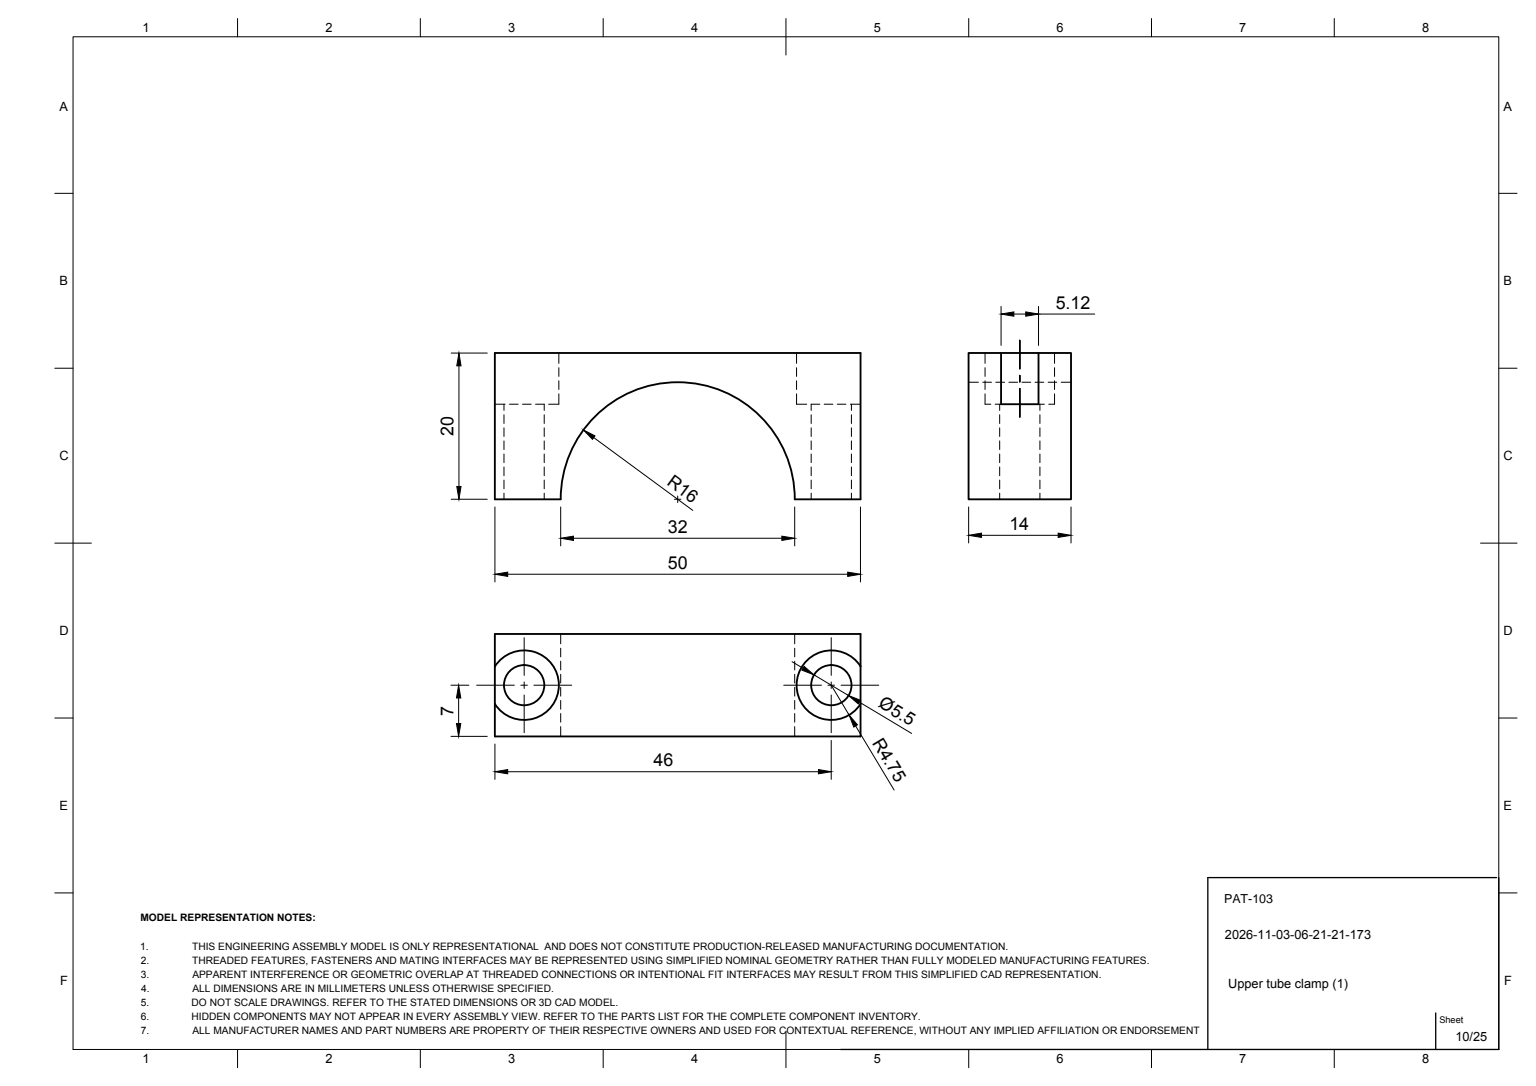
ISO-10303-21;
HEADER;
/* Generated by software containing ST-Developer
 * from STEP Tools, Inc. (www.steptools.com) 
 */

FILE_DESCRIPTION(
/* description */ ('Telescoping shaft support with lock collar'),
/* implementation_level */ '2;1');

FILE_NAME(
/* name */ 'Upper tube clamp (1).step',
/* time_stamp */ '2026-10-27T10:48:51-07:00',
/* author */ (''),
/* organization */ (''),
/* preprocessor_version */ 'ST-DEVELOPER v20.2',
/* originating_system */ 'Autodesk Translation Framework v15.17.0.0',
/* authorisation */ '');

FILE_SCHEMA (('AUTOMOTIVE_DESIGN { 1 0 10303 214 3 1 1 }'));
ENDSEC;

DATA;
#10=MECHANICAL_DESIGN_GEOMETRIC_PRESENTATION_REPRESENTATION('',(#246),#7349);
#206=SHAPE_REPRESENTATION_RELATIONSHIP('SRR','None',#7448,#226);
#226=ADVANCED_BREP_SHAPE_REPRESENTATION('',(#266),#7332);
#246=STYLED_ITEM('',(#7641),#266);
#266=MANIFOLD_SOLID_BREP('Body1',#3969);
#309=FACE_BOUND('',#828,.T.);
#310=FACE_BOUND('',#831,.T.);
#311=FACE_BOUND('',#840,.T.);
#312=FACE_BOUND('',#844,.T.);
#406=PLANE('',#4373);
#407=PLANE('',#4378);
#408=PLANE('',#4383);
#409=PLANE('',#4384);
#410=PLANE('',#4392);
#411=PLANE('',#4393);
#412=PLANE('',#4394);
#413=PLANE('',#4395);
#414=PLANE('',#4396);
#571=FACE_OUTER_BOUND('',#827,.T.);
#572=FACE_OUTER_BOUND('',#829,.T.);
#573=FACE_OUTER_BOUND('',#830,.T.);
#574=FACE_OUTER_BOUND('',#832,.T.);
#575=FACE_OUTER_BOUND('',#833,.T.);
#576=FACE_OUTER_BOUND('',#834,.T.);
#577=FACE_OUTER_BOUND('',#835,.T.);
#578=FACE_OUTER_BOUND('',#836,.T.);
#579=FACE_OUTER_BOUND('',#837,.T.);
#580=FACE_OUTER_BOUND('',#838,.T.);
#581=FACE_OUTER_BOUND('',#839,.T.);
#582=FACE_OUTER_BOUND('',#841,.T.);
#583=FACE_OUTER_BOUND('',#842,.T.);
#584=FACE_OUTER_BOUND('',#843,.T.);
#827=EDGE_LOOP('',(#3014,#3015));
#828=EDGE_LOOP('',(#3016));
#829=EDGE_LOOP('',(#3017,#3018,#3019,#3020));
#830=EDGE_LOOP('',(#3021,#3022));
#831=EDGE_LOOP('',(#3023));
#832=EDGE_LOOP('',(#3024,#3025,#3026,#3027));
#833=EDGE_LOOP('',(#3028,#3029,#3030,#3031,#3032,#3033,#3034,#3035));
#834=EDGE_LOOP('',(#3036,#3037,#3038,#3039,#3040,#3041,#3042,#3043));
#835=EDGE_LOOP('',(#3044,#3045,#3046,#3047));
#836=EDGE_LOOP('',(#3048,#3049,#3050,#3051));
#837=EDGE_LOOP('',(#3052,#3053,#3054,#3055));
#838=EDGE_LOOP('',(#3056,#3057,#3058,#3059,#3060,#3061));
#839=EDGE_LOOP('',(#3062,#3063,#3064,#3065));
#840=EDGE_LOOP('',(#3066));
#841=EDGE_LOOP('',(#3067,#3068,#3069,#3070,#3071,#3072));
#842=EDGE_LOOP('',(#3073,#3074,#3075,#3076,#3077,#3078,#3079,#3080));
#843=EDGE_LOOP('',(#3081,#3082,#3083,#3084));
#844=EDGE_LOOP('',(#3085));
#1131=LINE('',#6384,#1411);
#1132=LINE('',#6390,#1412);
#1133=LINE('',#6393,#1413);
#1134=LINE('',#6397,#1414);
#1135=LINE('',#6403,#1415);
#1136=LINE('',#6406,#1416);
#1137=LINE('',#6409,#1417);
#1138=LINE('',#6411,#1418);
#1139=LINE('',#6413,#1419);
#1140=LINE('',#6415,#1420);
#1141=LINE('',#6416,#1421);
#1142=LINE('',#6419,#1422);
#1143=LINE('',#6421,#1423);
#1144=LINE('',#6423,#1424);
#1145=LINE('',#6425,#1425);
#1146=LINE('',#6426,#1426);
#1147=LINE('',#6430,#1427);
#1148=LINE('',#6434,#1428);
#1149=LINE('',#6440,#1429);
#1150=LINE('',#6443,#1430);
#1151=LINE('',#6445,#1431);
#1152=LINE('',#6446,#1432);
#1153=LINE('',#6447,#1433);
#1154=LINE('',#6449,#1434);
#1155=LINE('',#6451,#1435);
#1156=LINE('',#6452,#1436);
#1411=VECTOR('',#5145,1.);
#1412=VECTOR('',#5152,1.);
#1413=VECTOR('',#5155,1.);
#1414=VECTOR('',#5158,1.);
#1415=VECTOR('',#5165,1.);
#1416=VECTOR('',#5168,1.);
#1417=VECTOR('',#5171,1.);
#1418=VECTOR('',#5172,1.);
#1419=VECTOR('',#5173,1.);
#1420=VECTOR('',#5174,1.);
#1421=VECTOR('',#5175,1.);
#1422=VECTOR('',#5178,1.);
#1423=VECTOR('',#5179,1.);
#1424=VECTOR('',#5180,1.);
#1425=VECTOR('',#5181,1.);
#1426=VECTOR('',#5182,1.);
#1427=VECTOR('',#5187,0.274999999999999);
#1428=VECTOR('',#5192,0.274999999999999);
#1429=VECTOR('',#5197,1.);
#1430=VECTOR('',#5200,1.);
#1431=VECTOR('',#5203,1.);
#1432=VECTOR('',#5204,1.);
#1433=VECTOR('',#5205,1.);
#1434=VECTOR('',#5208,1.);
#1435=VECTOR('',#5211,1.);
#1436=VECTOR('',#5212,1.);
#1669=CIRCLE('',#4374,0.475000000000001);
#1670=CIRCLE('',#4375,0.274999999999999);
#1671=CIRCLE('',#4377,0.475000000000001);
#1672=CIRCLE('',#4379,0.475000000000001);
#1673=CIRCLE('',#4380,0.274999999999999);
#1674=CIRCLE('',#4382,0.475000000000001);
#1675=CIRCLE('',#4386,0.274999999999999);
#1676=CIRCLE('',#4388,0.274999999999999);
#1677=CIRCLE('',#4390,1.6);
#1678=CIRCLE('',#4391,1.6);
#1922=VERTEX_POINT('',#6382);
#1923=VERTEX_POINT('',#6383);
#1924=VERTEX_POINT('',#6386);
#1925=VERTEX_POINT('',#6389);
#1926=VERTEX_POINT('',#6391);
#1927=VERTEX_POINT('',#6395);
#1928=VERTEX_POINT('',#6396);
#1929=VERTEX_POINT('',#6399);
#1930=VERTEX_POINT('',#6402);
#1931=VERTEX_POINT('',#6404);
#1932=VERTEX_POINT('',#6408);
#1933=VERTEX_POINT('',#6410);
#1934=VERTEX_POINT('',#6412);
#1935=VERTEX_POINT('',#6414);
#1936=VERTEX_POINT('',#6418);
#1937=VERTEX_POINT('',#6420);
#1938=VERTEX_POINT('',#6422);
#1939=VERTEX_POINT('',#6424);
#1940=VERTEX_POINT('',#6428);
#1941=VERTEX_POINT('',#6432);
#1942=VERTEX_POINT('',#6436);
#1943=VERTEX_POINT('',#6437);
#1944=VERTEX_POINT('',#6439);
#1945=VERTEX_POINT('',#6441);
#2319=EDGE_CURVE('',#1922,#1923,#1131,.T.);
#2320=EDGE_CURVE('',#1922,#1923,#1669,.T.);
#2321=EDGE_CURVE('',#1924,#1924,#1670,.T.);
#2322=EDGE_CURVE('',#1925,#1922,#1132,.T.);
#2323=EDGE_CURVE('',#1926,#1925,#1671,.T.);
#2324=EDGE_CURVE('',#1923,#1926,#1133,.T.);
#2325=EDGE_CURVE('',#1927,#1928,#1134,.T.);
#2326=EDGE_CURVE('',#1927,#1928,#1672,.T.);
#2327=EDGE_CURVE('',#1929,#1929,#1673,.T.);
#2328=EDGE_CURVE('',#1930,#1927,#1135,.T.);
#2329=EDGE_CURVE('',#1931,#1930,#1674,.T.);
#2330=EDGE_CURVE('',#1928,#1931,#1136,.T.);
#2331=EDGE_CURVE('',#1932,#1926,#1137,.T.);
#2332=EDGE_CURVE('',#1933,#1932,#1138,.T.);
#2333=EDGE_CURVE('',#1933,#1934,#1139,.T.);
#2334=EDGE_CURVE('',#1934,#1935,#1140,.T.);
#2335=EDGE_CURVE('',#1925,#1935,#1141,.T.);
#2336=EDGE_CURVE('',#1936,#1931,#1142,.T.);
#2337=EDGE_CURVE('',#1937,#1936,#1143,.T.);
#2338=EDGE_CURVE('',#1937,#1938,#1144,.T.);
#2339=EDGE_CURVE('',#1938,#1939,#1145,.T.);
#2340=EDGE_CURVE('',#1930,#1939,#1146,.T.);
#2341=EDGE_CURVE('',#1940,#1940,#1675,.T.);
#2342=EDGE_CURVE('',#1940,#1924,#1147,.T.);
#2343=EDGE_CURVE('',#1941,#1941,#1676,.T.);
#2344=EDGE_CURVE('',#1941,#1929,#1148,.T.);
#2345=EDGE_CURVE('',#1942,#1943,#1677,.T.);
#2346=EDGE_CURVE('',#1944,#1942,#1149,.T.);
#2347=EDGE_CURVE('',#1945,#1944,#1678,.T.);
#2348=EDGE_CURVE('',#1943,#1945,#1150,.T.);
#2349=EDGE_CURVE('',#1944,#1937,#1151,.T.);
#2350=EDGE_CURVE('',#1935,#1936,#1152,.T.);
#2351=EDGE_CURVE('',#1934,#1945,#1153,.T.);
#2352=EDGE_CURVE('',#1938,#1942,#1154,.T.);
#2353=EDGE_CURVE('',#1943,#1933,#1155,.T.);
#2354=EDGE_CURVE('',#1939,#1932,#1156,.T.);
#3014=ORIENTED_EDGE('',*,*,#2319,.F.);
#3015=ORIENTED_EDGE('',*,*,#2320,.T.);
#3016=ORIENTED_EDGE('',*,*,#2321,.F.);
#3017=ORIENTED_EDGE('',*,*,#2322,.F.);
#3018=ORIENTED_EDGE('',*,*,#2323,.F.);
#3019=ORIENTED_EDGE('',*,*,#2324,.F.);
#3020=ORIENTED_EDGE('',*,*,#2320,.F.);
#3021=ORIENTED_EDGE('',*,*,#2325,.F.);
#3022=ORIENTED_EDGE('',*,*,#2326,.T.);
#3023=ORIENTED_EDGE('',*,*,#2327,.F.);
#3024=ORIENTED_EDGE('',*,*,#2328,.F.);
#3025=ORIENTED_EDGE('',*,*,#2329,.F.);
#3026=ORIENTED_EDGE('',*,*,#2330,.F.);
#3027=ORIENTED_EDGE('',*,*,#2326,.F.);
#3028=ORIENTED_EDGE('',*,*,#2322,.T.);
#3029=ORIENTED_EDGE('',*,*,#2319,.T.);
#3030=ORIENTED_EDGE('',*,*,#2324,.T.);
#3031=ORIENTED_EDGE('',*,*,#2331,.F.);
#3032=ORIENTED_EDGE('',*,*,#2332,.F.);
#3033=ORIENTED_EDGE('',*,*,#2333,.T.);
#3034=ORIENTED_EDGE('',*,*,#2334,.T.);
#3035=ORIENTED_EDGE('',*,*,#2335,.F.);
#3036=ORIENTED_EDGE('',*,*,#2328,.T.);
#3037=ORIENTED_EDGE('',*,*,#2325,.T.);
#3038=ORIENTED_EDGE('',*,*,#2330,.T.);
#3039=ORIENTED_EDGE('',*,*,#2336,.F.);
#3040=ORIENTED_EDGE('',*,*,#2337,.F.);
#3041=ORIENTED_EDGE('',*,*,#2338,.T.);
#3042=ORIENTED_EDGE('',*,*,#2339,.T.);
#3043=ORIENTED_EDGE('',*,*,#2340,.F.);
#3044=ORIENTED_EDGE('',*,*,#2341,.F.);
#3045=ORIENTED_EDGE('',*,*,#2342,.T.);
#3046=ORIENTED_EDGE('',*,*,#2321,.T.);
#3047=ORIENTED_EDGE('',*,*,#2342,.F.);
#3048=ORIENTED_EDGE('',*,*,#2343,.F.);
#3049=ORIENTED_EDGE('',*,*,#2344,.T.);
#3050=ORIENTED_EDGE('',*,*,#2327,.T.);
#3051=ORIENTED_EDGE('',*,*,#2344,.F.);
#3052=ORIENTED_EDGE('',*,*,#2345,.F.);
#3053=ORIENTED_EDGE('',*,*,#2346,.F.);
#3054=ORIENTED_EDGE('',*,*,#2347,.F.);
#3055=ORIENTED_EDGE('',*,*,#2348,.F.);
#3056=ORIENTED_EDGE('',*,*,#2347,.T.);
#3057=ORIENTED_EDGE('',*,*,#2349,.T.);
#3058=ORIENTED_EDGE('',*,*,#2337,.T.);
#3059=ORIENTED_EDGE('',*,*,#2350,.F.);
#3060=ORIENTED_EDGE('',*,*,#2334,.F.);
#3061=ORIENTED_EDGE('',*,*,#2351,.T.);
#3062=ORIENTED_EDGE('',*,*,#2346,.T.);
#3063=ORIENTED_EDGE('',*,*,#2352,.F.);
#3064=ORIENTED_EDGE('',*,*,#2338,.F.);
#3065=ORIENTED_EDGE('',*,*,#2349,.F.);
#3066=ORIENTED_EDGE('',*,*,#2343,.T.);
#3067=ORIENTED_EDGE('',*,*,#2345,.T.);
#3068=ORIENTED_EDGE('',*,*,#2353,.T.);
#3069=ORIENTED_EDGE('',*,*,#2332,.T.);
#3070=ORIENTED_EDGE('',*,*,#2354,.F.);
#3071=ORIENTED_EDGE('',*,*,#2339,.F.);
#3072=ORIENTED_EDGE('',*,*,#2352,.T.);
#3073=ORIENTED_EDGE('',*,*,#2323,.T.);
#3074=ORIENTED_EDGE('',*,*,#2335,.T.);
#3075=ORIENTED_EDGE('',*,*,#2350,.T.);
#3076=ORIENTED_EDGE('',*,*,#2336,.T.);
#3077=ORIENTED_EDGE('',*,*,#2329,.T.);
#3078=ORIENTED_EDGE('',*,*,#2340,.T.);
#3079=ORIENTED_EDGE('',*,*,#2354,.T.);
#3080=ORIENTED_EDGE('',*,*,#2331,.T.);
#3081=ORIENTED_EDGE('',*,*,#2348,.T.);
#3082=ORIENTED_EDGE('',*,*,#2351,.F.);
#3083=ORIENTED_EDGE('',*,*,#2333,.F.);
#3084=ORIENTED_EDGE('',*,*,#2353,.F.);
#3085=ORIENTED_EDGE('',*,*,#2341,.T.);
#3689=CYLINDRICAL_SURFACE('',#4376,0.475000000000001);
#3690=CYLINDRICAL_SURFACE('',#4381,0.475000000000001);
#3691=CYLINDRICAL_SURFACE('',#4385,0.274999999999999);
#3692=CYLINDRICAL_SURFACE('',#4387,0.274999999999999);
#3693=CYLINDRICAL_SURFACE('',#4389,1.6);
#3814=ADVANCED_FACE('',(#571,#309),#406,.T.);
#3815=ADVANCED_FACE('',(#572),#3689,.F.);
#3816=ADVANCED_FACE('',(#573,#310),#407,.T.);
#3817=ADVANCED_FACE('',(#574),#3690,.F.);
#3818=ADVANCED_FACE('',(#575),#408,.T.);
#3819=ADVANCED_FACE('',(#576),#409,.T.);
#3820=ADVANCED_FACE('',(#577),#3691,.F.);
#3821=ADVANCED_FACE('',(#578),#3692,.F.);
#3822=ADVANCED_FACE('',(#579),#3693,.F.);
#3823=ADVANCED_FACE('',(#580),#410,.T.);
#3824=ADVANCED_FACE('',(#581,#311),#411,.F.);
#3825=ADVANCED_FACE('',(#582),#412,.T.);
#3826=ADVANCED_FACE('',(#583),#413,.T.);
#3827=ADVANCED_FACE('',(#584,#312),#414,.F.);
#3969=CLOSED_SHELL('',(#3814,#3815,#3816,#3817,#3818,#3819,#3820,#3821,
#3822,#3823,#3824,#3825,#3826,#3827));
#4372=AXIS2_PLACEMENT_3D('',#6380,#5141,#5142);
#4373=AXIS2_PLACEMENT_3D('',#6381,#5143,#5144);
#4374=AXIS2_PLACEMENT_3D('',#6385,#5146,#5147);
#4375=AXIS2_PLACEMENT_3D('',#6387,#5148,#5149);
#4376=AXIS2_PLACEMENT_3D('',#6388,#5150,#5151);
#4377=AXIS2_PLACEMENT_3D('',#6392,#5153,#5154);
#4378=AXIS2_PLACEMENT_3D('',#6394,#5156,#5157);
#4379=AXIS2_PLACEMENT_3D('',#6398,#5159,#5160);
#4380=AXIS2_PLACEMENT_3D('',#6400,#5161,#5162);
#4381=AXIS2_PLACEMENT_3D('',#6401,#5163,#5164);
#4382=AXIS2_PLACEMENT_3D('',#6405,#5166,#5167);
#4383=AXIS2_PLACEMENT_3D('',#6407,#5169,#5170);
#4384=AXIS2_PLACEMENT_3D('',#6417,#5176,#5177);
#4385=AXIS2_PLACEMENT_3D('',#6427,#5183,#5184);
#4386=AXIS2_PLACEMENT_3D('',#6429,#5185,#5186);
#4387=AXIS2_PLACEMENT_3D('',#6431,#5188,#5189);
#4388=AXIS2_PLACEMENT_3D('',#6433,#5190,#5191);
#4389=AXIS2_PLACEMENT_3D('',#6435,#5193,#5194);
#4390=AXIS2_PLACEMENT_3D('',#6438,#5195,#5196);
#4391=AXIS2_PLACEMENT_3D('',#6442,#5198,#5199);
#4392=AXIS2_PLACEMENT_3D('',#6444,#5201,#5202);
#4393=AXIS2_PLACEMENT_3D('',#6448,#5206,#5207);
#4394=AXIS2_PLACEMENT_3D('',#6450,#5209,#5210);
#4395=AXIS2_PLACEMENT_3D('',#6453,#5213,#5214);
#4396=AXIS2_PLACEMENT_3D('',#6454,#5215,#5216);
#5141=DIRECTION('axis',(0.,0.,1.));
#5142=DIRECTION('refdir',(1.,0.,0.));
#5143=DIRECTION('center_axis',(0.,0.,1.));
#5144=DIRECTION('ref_axis',(1.,0.,0.));
#5145=DIRECTION('',(-1.,0.,0.));
#5146=DIRECTION('center_axis',(0.,0.,1.));
#5147=DIRECTION('ref_axis',(1.,0.,0.));
#5148=DIRECTION('center_axis',(0.,0.,1.));
#5149=DIRECTION('ref_axis',(1.,0.,0.));
#5150=DIRECTION('center_axis',(0.,0.,1.));
#5151=DIRECTION('ref_axis',(5.0532154980743E-16,1.,0.));
#5152=DIRECTION('',(0.,0.,-1.));
#5153=DIRECTION('center_axis',(0.,0.,-1.));
#5154=DIRECTION('ref_axis',(1.,0.,0.));
#5155=DIRECTION('',(0.,0.,1.));
#5156=DIRECTION('center_axis',(0.,0.,1.));
#5157=DIRECTION('ref_axis',(1.,0.,0.));
#5158=DIRECTION('',(1.,0.,0.));
#5159=DIRECTION('center_axis',(0.,0.,1.));
#5160=DIRECTION('ref_axis',(1.,0.,0.));
#5161=DIRECTION('center_axis',(0.,0.,1.));
#5162=DIRECTION('ref_axis',(1.,0.,0.));
#5163=DIRECTION('center_axis',(0.,0.,1.));
#5164=DIRECTION('ref_axis',(-1.83697019872103E-16,-1.,0.));
#5165=DIRECTION('',(0.,0.,-1.));
#5166=DIRECTION('center_axis',(0.,0.,-1.));
#5167=DIRECTION('ref_axis',(1.,0.,0.));
#5168=DIRECTION('',(0.,0.,1.));
#5169=DIRECTION('center_axis',(0.,-1.,0.));
#5170=DIRECTION('ref_axis',(1.,0.,0.));
#5171=DIRECTION('',(1.,0.,0.));
#5172=DIRECTION('',(0.,0.,1.));
#5173=DIRECTION('',(1.,0.,0.));
#5174=DIRECTION('',(0.,0.,1.));
#5175=DIRECTION('',(1.,0.,0.));
#5176=DIRECTION('center_axis',(0.,1.,0.));
#5177=DIRECTION('ref_axis',(-1.,0.,0.));
#5178=DIRECTION('',(-1.,0.,0.));
#5179=DIRECTION('',(0.,0.,1.));
#5180=DIRECTION('',(-1.,0.,0.));
#5181=DIRECTION('',(0.,0.,1.));
#5182=DIRECTION('',(-1.,0.,0.));
#5183=DIRECTION('center_axis',(0.,0.,1.));
#5184=DIRECTION('ref_axis',(1.,0.,0.));
#5185=DIRECTION('center_axis',(0.,0.,1.));
#5186=DIRECTION('ref_axis',(1.,0.,0.));
#5187=DIRECTION('',(0.,0.,1.));
#5188=DIRECTION('center_axis',(0.,0.,1.));
#5189=DIRECTION('ref_axis',(1.,0.,0.));
#5190=DIRECTION('center_axis',(0.,0.,1.));
#5191=DIRECTION('ref_axis',(1.,0.,0.));
#5192=DIRECTION('',(0.,0.,1.));
#5193=DIRECTION('center_axis',(1.,0.,0.));
#5194=DIRECTION('ref_axis',(0.,1.22464679914735E-16,1.));
#5195=DIRECTION('center_axis',(1.,0.,0.));
#5196=DIRECTION('ref_axis',(0.,0.,-1.));
#5197=DIRECTION('',(-1.,0.,0.));
#5198=DIRECTION('center_axis',(-1.,0.,0.));
#5199=DIRECTION('ref_axis',(0.,0.,-1.));
#5200=DIRECTION('',(1.,0.,0.));
#5201=DIRECTION('center_axis',(1.,0.,0.));
#5202=DIRECTION('ref_axis',(0.,1.,0.));
#5203=DIRECTION('',(0.,1.,0.));
#5204=DIRECTION('',(0.,1.,0.));
#5205=DIRECTION('',(0.,1.,0.));
#5206=DIRECTION('center_axis',(0.,0.,1.));
#5207=DIRECTION('ref_axis',(1.,0.,0.));
#5208=DIRECTION('',(0.,-1.,0.));
#5209=DIRECTION('center_axis',(-1.,0.,0.));
#5210=DIRECTION('ref_axis',(0.,-1.,0.));
#5211=DIRECTION('',(0.,-1.,0.));
#5212=DIRECTION('',(0.,-1.,0.));
#5213=DIRECTION('center_axis',(0.,0.,1.));
#5214=DIRECTION('ref_axis',(1.,0.,0.));
#5215=DIRECTION('center_axis',(0.,0.,1.));
#5216=DIRECTION('ref_axis',(1.,0.,0.));
#6380=CARTESIAN_POINT('',(0.,0.,0.));
#6381=CARTESIAN_POINT('Origin',(7.8,-2.1,4.8));
#6382=CARTESIAN_POINT('',(8.05617376914899,-2.5,4.8));
#6383=CARTESIAN_POINT('',(7.54382623085101,-2.5,4.8));
#6384=CARTESIAN_POINT('',(7.45,-2.5,4.8));
#6385=CARTESIAN_POINT('Origin',(7.8,-2.1,4.8));
#6386=CARTESIAN_POINT('',(7.525,-2.1,4.8));
#6387=CARTESIAN_POINT('Origin',(7.8,-2.1,4.8));
#6388=CARTESIAN_POINT('Origin',(7.8,-2.1,4.8));
#6389=CARTESIAN_POINT('',(8.05617376914899,-2.5,5.5));
#6390=CARTESIAN_POINT('',(8.05617376914899,-2.5,4.8));
#6391=CARTESIAN_POINT('',(7.54382623085101,-2.5,5.5));
#6392=CARTESIAN_POINT('Origin',(7.8,-2.1,5.5));
#6393=CARTESIAN_POINT('',(7.54382623085101,-2.5,4.8));
#6394=CARTESIAN_POINT('Origin',(7.8,2.1,4.8));
#6395=CARTESIAN_POINT('',(7.54382623085101,2.5,4.8));
#6396=CARTESIAN_POINT('',(8.05617376914899,2.5,4.8));
#6397=CARTESIAN_POINT('',(8.15,2.5,4.8));
#6398=CARTESIAN_POINT('Origin',(7.8,2.1,4.8));
#6399=CARTESIAN_POINT('',(7.525,2.1,4.8));
#6400=CARTESIAN_POINT('Origin',(7.8,2.1,4.8));
#6401=CARTESIAN_POINT('Origin',(7.8,2.1,4.8));
#6402=CARTESIAN_POINT('',(7.54382623085101,2.5,5.5));
#6403=CARTESIAN_POINT('',(7.54382623085101,2.5,4.8));
#6404=CARTESIAN_POINT('',(8.05617376914899,2.5,5.5));
#6405=CARTESIAN_POINT('Origin',(7.8,2.1,5.5));
#6406=CARTESIAN_POINT('',(8.05617376914899,2.5,4.8));
#6407=CARTESIAN_POINT('Origin',(7.1,-2.5,3.5));
#6408=CARTESIAN_POINT('',(7.1,-2.5,5.5));
#6409=CARTESIAN_POINT('',(7.1,-2.5,5.5));
#6410=CARTESIAN_POINT('',(7.1,-2.5,3.5));
#6411=CARTESIAN_POINT('',(7.1,-2.5,3.5));
#6412=CARTESIAN_POINT('',(8.5,-2.5,3.5));
#6413=CARTESIAN_POINT('',(7.1,-2.5,3.5));
#6414=CARTESIAN_POINT('',(8.5,-2.5,5.5));
#6415=CARTESIAN_POINT('',(8.5,-2.5,3.5));
#6416=CARTESIAN_POINT('',(7.1,-2.5,5.5));
#6417=CARTESIAN_POINT('Origin',(8.5,2.5,3.5));
#6418=CARTESIAN_POINT('',(8.5,2.5,5.5));
#6419=CARTESIAN_POINT('',(8.5,2.5,5.5));
#6420=CARTESIAN_POINT('',(8.5,2.5,3.5));
#6421=CARTESIAN_POINT('',(8.5,2.5,3.5));
#6422=CARTESIAN_POINT('',(7.1,2.5,3.5));
#6423=CARTESIAN_POINT('',(8.5,2.5,3.5));
#6424=CARTESIAN_POINT('',(7.1,2.5,5.5));
#6425=CARTESIAN_POINT('',(7.1,2.5,3.5));
#6426=CARTESIAN_POINT('',(8.5,2.5,5.5));
#6427=CARTESIAN_POINT('Origin',(7.8,-2.1,3.4));
#6428=CARTESIAN_POINT('',(7.525,-2.1,3.5));
#6429=CARTESIAN_POINT('Origin',(7.8,-2.1,3.5));
#6430=CARTESIAN_POINT('',(7.525,-2.1,3.4));
#6431=CARTESIAN_POINT('Origin',(7.8,2.1,3.4));
#6432=CARTESIAN_POINT('',(7.525,2.1,3.5));
#6433=CARTESIAN_POINT('Origin',(7.8,2.1,3.5));
#6434=CARTESIAN_POINT('',(7.525,2.1,3.4));
#6435=CARTESIAN_POINT('Origin',(7.,0.,3.5));
#6436=CARTESIAN_POINT('',(7.1,1.6,3.5));
#6437=CARTESIAN_POINT('',(7.1,-1.6,3.5));
#6438=CARTESIAN_POINT('Origin',(7.1,0.,3.5));
#6439=CARTESIAN_POINT('',(8.5,1.6,3.5));
#6440=CARTESIAN_POINT('',(7.,1.6,3.5));
#6441=CARTESIAN_POINT('',(8.5,-1.6,3.5));
#6442=CARTESIAN_POINT('Origin',(8.5,0.,3.5));
#6443=CARTESIAN_POINT('',(7.,-1.6,3.5));
#6444=CARTESIAN_POINT('Origin',(8.5,-2.5,3.5));
#6445=CARTESIAN_POINT('',(8.5,-2.5,3.5));
#6446=CARTESIAN_POINT('',(8.5,-2.5,5.5));
#6447=CARTESIAN_POINT('',(8.5,-2.5,3.5));
#6448=CARTESIAN_POINT('Origin',(7.8,0.,3.5));
#6449=CARTESIAN_POINT('',(7.1,2.5,3.5));
#6450=CARTESIAN_POINT('Origin',(7.1,2.5,3.5));
#6451=CARTESIAN_POINT('',(7.1,2.5,3.5));
#6452=CARTESIAN_POINT('',(7.1,2.5,5.5));
#6453=CARTESIAN_POINT('Origin',(7.8,0.,5.5));
#6454=CARTESIAN_POINT('Origin',(7.8,0.,3.5));
#7307=UNCERTAINTY_MEASURE_WITH_UNIT(LENGTH_MEASURE(0.001),#7350,
'DISTANCE_ACCURACY_VALUE',
'Maximum model space distance between geometric entities at asserted c
onnectivities');
#7324=UNCERTAINTY_MEASURE_WITH_UNIT(LENGTH_MEASURE(0.001),#7350,
'DISTANCE_ACCURACY_VALUE',
'Maximum model space distance between geometric entities at asserted c
onnectivities');
#7332=(
GEOMETRIC_REPRESENTATION_CONTEXT(3)
GLOBAL_UNCERTAINTY_ASSIGNED_CONTEXT((#7307))
GLOBAL_UNIT_ASSIGNED_CONTEXT((#7350,#7352,#7353))
REPRESENTATION_CONTEXT('','3D')
);
#7349=(
GEOMETRIC_REPRESENTATION_CONTEXT(3)
GLOBAL_UNCERTAINTY_ASSIGNED_CONTEXT((#7324))
GLOBAL_UNIT_ASSIGNED_CONTEXT((#7350,#7352,#7353))
REPRESENTATION_CONTEXT('','3D')
);
#7350=(
LENGTH_UNIT()
NAMED_UNIT(*)
SI_UNIT(.CENTI.,.METRE.)
);
#7352=(
NAMED_UNIT(*)
PLANE_ANGLE_UNIT()
SI_UNIT($,.RADIAN.)
);
#7353=(
NAMED_UNIT(*)
SI_UNIT($,.STERADIAN.)
SOLID_ANGLE_UNIT()
);
#7361=SHAPE_DEFINITION_REPRESENTATION(#7385,#7448);
#7385=PRODUCT_DEFINITION_SHAPE('',$,#7473);
#7448=SHAPE_REPRESENTATION('',(#4372),#7332);
#7465=PRODUCT_DEFINITION_CONTEXT('part definition',#7539,'design');
#7473=PRODUCT_DEFINITION('Upper tube clamp (1)','Upper tube clamp (1)',#7497,
#7465);
#7497=PRODUCT_DEFINITION_FORMATION('',$,#7548);
#7539=APPLICATION_CONTEXT(
'Core Data for Automotive Mechanical Design Process');
#7540=PRODUCT_CONTEXT('part definition',#7539,'mechanical');
#7548=PRODUCT('Upper tube clamp (1)','Upper tube clamp (1)',
'Upper tube clamp (1)',(#7540));
#7635=COLOUR_RGB('Off White',0.89,0.88,0.83);
#7636=FILL_AREA_STYLE_COLOUR('',#7635);
#7637=FILL_AREA_STYLE('',(#7636));
#7638=SURFACE_STYLE_FILL_AREA(#7637);
#7639=SURFACE_SIDE_STYLE('',(#7638));
#7640=SURFACE_STYLE_USAGE(.BOTH.,#7639);
#7641=PRESENTATION_STYLE_ASSIGNMENT((#7640));
ENDSEC;
END-ISO-10303-21;
